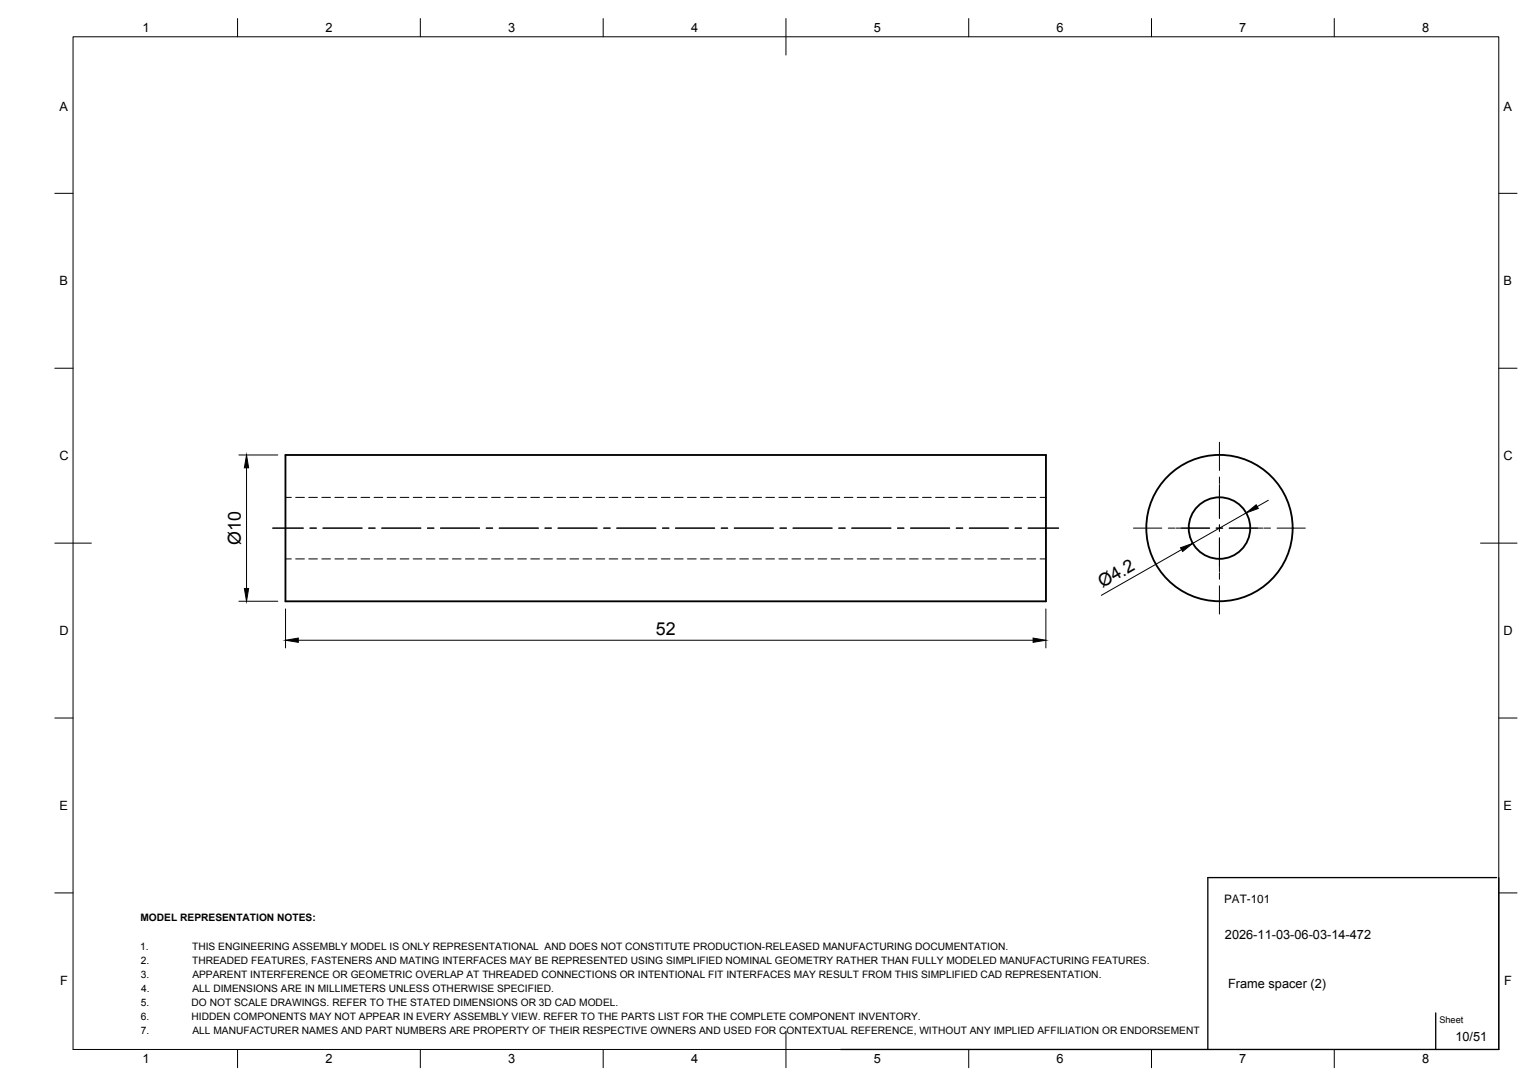
ISO-10303-21;
HEADER;
/* Generated by software containing ST-Developer
 * from STEP Tools, Inc. (www.steptools.com) 
 */

FILE_DESCRIPTION(
/* description */ ('Spur gear reduction stage 2-1 on bearing plates'),
/* implementation_level */ '2;1');

FILE_NAME(
/* name */ 'Frame spacer (2).step',
/* time_stamp */ '2026-10-28T03:22:07-07:00',
/* author */ (''),
/* organization */ (''),
/* preprocessor_version */ 'ST-DEVELOPER v20.2',
/* originating_system */ 'Autodesk Translation Framework v15.17.0.0',
/* authorisation */ '');

FILE_SCHEMA (('AUTOMOTIVE_DESIGN { 1 0 10303 214 3 1 1 }'));
ENDSEC;

DATA;
#10=MECHANICAL_DESIGN_GEOMETRIC_PRESENTATION_REPRESENTATION('',(#952),#53909);
#866=SHAPE_REPRESENTATION_RELATIONSHIP('SRR','None',#54093,#909);
#909=ADVANCED_BREP_SHAPE_REPRESENTATION('',(#1010),#53867);
#952=STYLED_ITEM('',(#54376),#1010);
#1010=MANIFOLD_SOLID_BREP('Body1',#11276);
#1136=FACE_BOUND('',#2316,.T.);
#1137=FACE_BOUND('',#2318,.T.);
#1276=PLANE('',#12002);
#1277=PLANE('',#12003);
#1589=FACE_OUTER_BOUND('',#2313,.T.);
#1590=FACE_OUTER_BOUND('',#2314,.T.);
#1591=FACE_OUTER_BOUND('',#2315,.T.);
#1592=FACE_OUTER_BOUND('',#2317,.T.);
#2313=EDGE_LOOP('',(#7712,#7713,#7714,#7715));
#2314=EDGE_LOOP('',(#7716,#7717,#7718,#7719));
#2315=EDGE_LOOP('',(#7720));
#2316=EDGE_LOOP('',(#7721));
#2317=EDGE_LOOP('',(#7722));
#2318=EDGE_LOOP('',(#7723));
#3061=LINE('',#16373,#3702);
#3062=LINE('',#16379,#3703);
#3702=VECTOR('',#13450,0.210000000000001);
#3703=VECTOR('',#13457,0.5);
#4355=CIRCLE('',#11997,0.210000000000001);
#4356=CIRCLE('',#11998,0.210000000000001);
#4357=CIRCLE('',#12000,0.5);
#4358=CIRCLE('',#12001,0.5);
#4904=VERTEX_POINT('',#16370);
#4905=VERTEX_POINT('',#16372);
#4906=VERTEX_POINT('',#16376);
#4907=VERTEX_POINT('',#16378);
#5998=EDGE_CURVE('',#4904,#4904,#4355,.T.);
#5999=EDGE_CURVE('',#4904,#4905,#3061,.T.);
#6000=EDGE_CURVE('',#4905,#4905,#4356,.T.);
#6001=EDGE_CURVE('',#4906,#4906,#4357,.T.);
#6002=EDGE_CURVE('',#4906,#4907,#3062,.T.);
#6003=EDGE_CURVE('',#4907,#4907,#4358,.T.);
#7712=ORIENTED_EDGE('',*,*,#5998,.F.);
#7713=ORIENTED_EDGE('',*,*,#5999,.T.);
#7714=ORIENTED_EDGE('',*,*,#6000,.T.);
#7715=ORIENTED_EDGE('',*,*,#5999,.F.);
#7716=ORIENTED_EDGE('',*,*,#6001,.F.);
#7717=ORIENTED_EDGE('',*,*,#6002,.T.);
#7718=ORIENTED_EDGE('',*,*,#6003,.T.);
#7719=ORIENTED_EDGE('',*,*,#6002,.F.);
#7720=ORIENTED_EDGE('',*,*,#6001,.T.);
#7721=ORIENTED_EDGE('',*,*,#5998,.T.);
#7722=ORIENTED_EDGE('',*,*,#6003,.F.);
#7723=ORIENTED_EDGE('',*,*,#6000,.F.);
#10468=CYLINDRICAL_SURFACE('',#11996,0.210000000000001);
#10469=CYLINDRICAL_SURFACE('',#11999,0.5);
#10709=ADVANCED_FACE('',(#1589),#10468,.F.);
#10710=ADVANCED_FACE('',(#1590),#10469,.T.);
#10711=ADVANCED_FACE('',(#1591,#1136),#1276,.T.);
#10712=ADVANCED_FACE('',(#1592,#1137),#1277,.F.);
#11276=CLOSED_SHELL('',(#10709,#10710,#10711,#10712));
#11995=AXIS2_PLACEMENT_3D('',#16368,#13444,#13445);
#11996=AXIS2_PLACEMENT_3D('',#16369,#13446,#13447);
#11997=AXIS2_PLACEMENT_3D('',#16371,#13448,#13449);
#11998=AXIS2_PLACEMENT_3D('',#16374,#13451,#13452);
#11999=AXIS2_PLACEMENT_3D('',#16375,#13453,#13454);
#12000=AXIS2_PLACEMENT_3D('',#16377,#13455,#13456);
#12001=AXIS2_PLACEMENT_3D('',#16380,#13458,#13459);
#12002=AXIS2_PLACEMENT_3D('',#16381,#13460,#13461);
#12003=AXIS2_PLACEMENT_3D('',#16382,#13462,#13463);
#13444=DIRECTION('axis',(0.,0.,1.));
#13445=DIRECTION('refdir',(1.,0.,0.));
#13446=DIRECTION('center_axis',(0.,1.,0.));
#13447=DIRECTION('ref_axis',(1.,0.,0.));
#13448=DIRECTION('center_axis',(0.,-1.,0.));
#13449=DIRECTION('ref_axis',(1.,0.,0.));
#13450=DIRECTION('',(0.,-1.,0.));
#13451=DIRECTION('center_axis',(0.,-1.,0.));
#13452=DIRECTION('ref_axis',(1.,0.,0.));
#13453=DIRECTION('center_axis',(0.,1.,0.));
#13454=DIRECTION('ref_axis',(1.,0.,0.));
#13455=DIRECTION('center_axis',(0.,1.,0.));
#13456=DIRECTION('ref_axis',(1.,0.,0.));
#13457=DIRECTION('',(0.,-1.,0.));
#13458=DIRECTION('center_axis',(0.,1.,0.));
#13459=DIRECTION('ref_axis',(1.,0.,0.));
#13460=DIRECTION('center_axis',(0.,1.,0.));
#13461=DIRECTION('ref_axis',(1.,0.,0.));
#13462=DIRECTION('center_axis',(0.,1.,0.));
#13463=DIRECTION('ref_axis',(1.,0.,0.));
#16368=CARTESIAN_POINT('',(0.,0.,0.));
#16369=CARTESIAN_POINT('Origin',(10.,-2.6,2.));
#16370=CARTESIAN_POINT('',(9.79,2.6,2.));
#16371=CARTESIAN_POINT('Origin',(10.,2.6,2.));
#16372=CARTESIAN_POINT('',(9.79,-2.6,2.));
#16373=CARTESIAN_POINT('',(9.79,-2.6,2.));
#16374=CARTESIAN_POINT('Origin',(10.,-2.6,2.));
#16375=CARTESIAN_POINT('Origin',(10.,-2.6,2.));
#16376=CARTESIAN_POINT('',(9.5,2.6,2.));
#16377=CARTESIAN_POINT('Origin',(10.,2.6,2.));
#16378=CARTESIAN_POINT('',(9.5,-2.6,2.));
#16379=CARTESIAN_POINT('',(9.5,-2.6,2.));
#16380=CARTESIAN_POINT('Origin',(10.,-2.6,2.));
#16381=CARTESIAN_POINT('Origin',(10.,2.6,2.));
#16382=CARTESIAN_POINT('Origin',(10.,-2.6,2.));
#53817=UNCERTAINTY_MEASURE_WITH_UNIT(LENGTH_MEASURE(0.001),#53910,
'DISTANCE_ACCURACY_VALUE',
'Maximum model space distance between geometric entities at asserted c
onnectivities');
#53859=UNCERTAINTY_MEASURE_WITH_UNIT(LENGTH_MEASURE(0.001),#53910,
'DISTANCE_ACCURACY_VALUE',
'Maximum model space distance between geometric entities at asserted c
onnectivities');
#53867=(
GEOMETRIC_REPRESENTATION_CONTEXT(3)
GLOBAL_UNCERTAINTY_ASSIGNED_CONTEXT((#53817))
GLOBAL_UNIT_ASSIGNED_CONTEXT((#53910,#53912,#53913))
REPRESENTATION_CONTEXT('','3D')
);
#53909=(
GEOMETRIC_REPRESENTATION_CONTEXT(3)
GLOBAL_UNCERTAINTY_ASSIGNED_CONTEXT((#53859))
GLOBAL_UNIT_ASSIGNED_CONTEXT((#53910,#53912,#53913))
REPRESENTATION_CONTEXT('','3D')
);
#53910=(
LENGTH_UNIT()
NAMED_UNIT(*)
SI_UNIT(.CENTI.,.METRE.)
);
#53912=(
NAMED_UNIT(*)
PLANE_ANGLE_UNIT()
SI_UNIT($,.RADIAN.)
);
#53913=(
NAMED_UNIT(*)
SI_UNIT($,.STERADIAN.)
SOLID_ANGLE_UNIT()
);
#53921=SHAPE_DEFINITION_REPRESENTATION(#53970,#54093);
#53970=PRODUCT_DEFINITION_SHAPE('',$,#54143);
#54093=SHAPE_REPRESENTATION('',(#11995),#53867);
#54135=PRODUCT_DEFINITION_CONTEXT('part definition',#54284,'design');
#54143=PRODUCT_DEFINITION('Frame spacer (2)','Frame spacer (2)',#54192,#54135);
#54192=PRODUCT_DEFINITION_FORMATION('',$,#54293);
#54284=APPLICATION_CONTEXT(
'Core Data for Automotive Mechanical Design Process');
#54285=PRODUCT_CONTEXT('part definition',#54284,'mechanical');
#54293=PRODUCT('Frame spacer (2)','Frame spacer (2)','Frame spacer (2)',(#54285));
#54370=COLOUR_RGB('Dark Blue',0.08,0.2,0.34);
#54371=FILL_AREA_STYLE_COLOUR('',#54370);
#54372=FILL_AREA_STYLE('',(#54371));
#54373=SURFACE_STYLE_FILL_AREA(#54372);
#54374=SURFACE_SIDE_STYLE('',(#54373));
#54375=SURFACE_STYLE_USAGE(.BOTH.,#54374);
#54376=PRESENTATION_STYLE_ASSIGNMENT((#54375));
ENDSEC;
END-ISO-10303-21;
